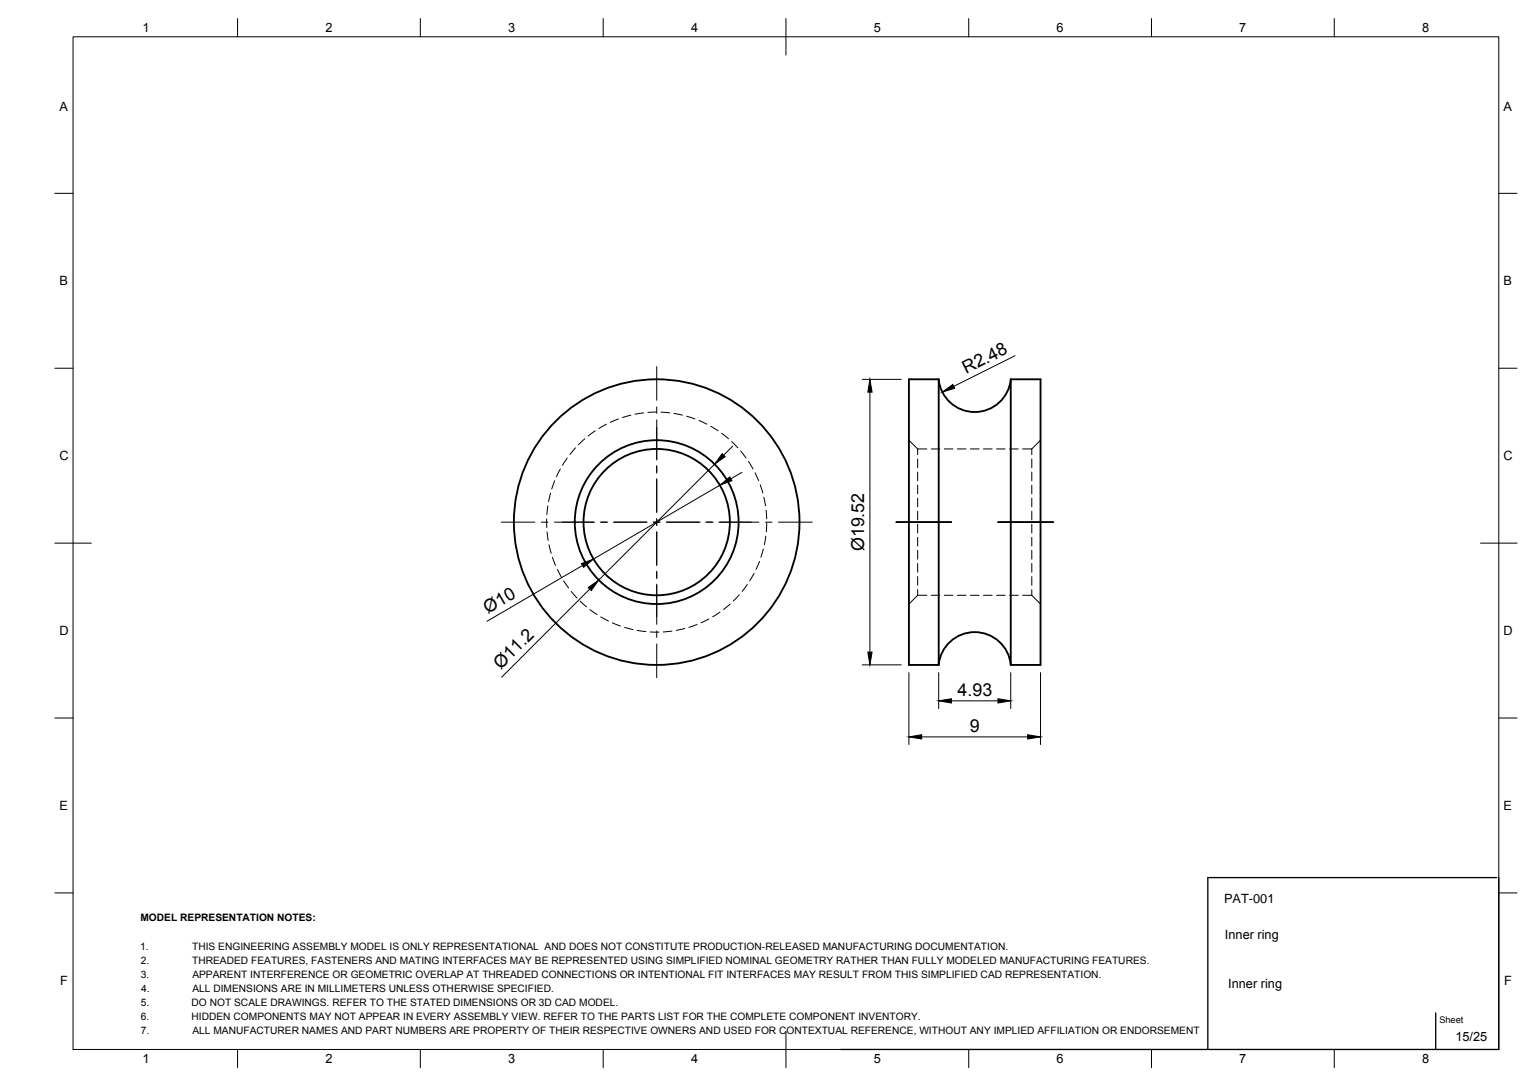
ISO-10303-21;
HEADER;
/* Generated by software containing ST-Developer
 * from STEP Tools, Inc. (www.steptools.com) 
 */

FILE_DESCRIPTION(
/* description */ ('PAT-001'),
/* implementation_level */ '2;1');

FILE_NAME(
/* name */ 'Inner ring.step',
/* time_stamp */ '2026-10-29T17:07:15-07:00',
/* author */ (''),
/* organization */ (''),
/* preprocessor_version */ 'ST-DEVELOPER v20.2',
/* originating_system */ 'Autodesk Translation Framework v15.17.0.0',
/* authorisation */ '');

FILE_SCHEMA (('AUTOMOTIVE_DESIGN { 1 0 10303 214 3 1 1 }'));
ENDSEC;

DATA;
#10=MECHANICAL_DESIGN_GEOMETRIC_PRESENTATION_REPRESENTATION('',(#378),#9622);
#305=CONICAL_SURFACE('',#5582,0.53,0.785398163397448);
#306=CONICAL_SURFACE('',#5589,0.53,0.785398163397448);
#321=TOROIDAL_SURFACE('',#5571,1.,0.247676);
#328=SHAPE_REPRESENTATION_RELATIONSHIP('SRR','None',#9752,#353);
#353=ADVANCED_BREP_SHAPE_REPRESENTATION('',(#411),#9601);
#378=STYLED_ITEM('',(#9962),#411);
#411=MANIFOLD_SOLID_BREP('Body1',#5203);
#449=FACE_BOUND('',#1055,.T.);
#450=FACE_BOUND('',#1058,.T.);
#542=PLANE('',#5584);
#543=PLANE('',#5587);
#742=FACE_OUTER_BOUND('',#1050,.T.);
#743=FACE_OUTER_BOUND('',#1051,.T.);
#744=FACE_OUTER_BOUND('',#1052,.T.);
#745=FACE_OUTER_BOUND('',#1053,.T.);
#746=FACE_OUTER_BOUND('',#1054,.T.);
#747=FACE_OUTER_BOUND('',#1056,.T.);
#748=FACE_OUTER_BOUND('',#1057,.T.);
#749=FACE_OUTER_BOUND('',#1059,.T.);
#1050=EDGE_LOOP('',(#3595,#3596,#3597,#3598,#3599,#3600));
#1051=EDGE_LOOP('',(#3601,#3602,#3603,#3604,#3605));
#1052=EDGE_LOOP('',(#3606,#3607,#3608,#3609));
#1053=EDGE_LOOP('',(#3610,#3611,#3612,#3613));
#1054=EDGE_LOOP('',(#3614));
#1055=EDGE_LOOP('',(#3615));
#1056=EDGE_LOOP('',(#3616,#3617,#3618,#3619,#3620));
#1057=EDGE_LOOP('',(#3621));
#1058=EDGE_LOOP('',(#3622));
#1059=EDGE_LOOP('',(#3623,#3624,#3625,#3626));
#1411=LINE('',#7821,#1816);
#1412=LINE('',#7827,#1817);
#1413=LINE('',#7831,#1818);
#1414=LINE('',#7837,#1819);
#1415=LINE('',#7842,#1820);
#1816=VECTOR('',#6258,0.976185);
#1817=VECTOR('',#6265,0.5);
#1818=VECTOR('',#6270,0.53);
#1819=VECTOR('',#6279,0.976185);
#1820=VECTOR('',#6286,0.53);
#2234=CIRCLE('',#5572,0.976185);
#2235=CIRCLE('',#5573,0.976185);
#2236=CIRCLE('',#5574,0.247676);
#2237=CIRCLE('',#5575,0.976185);
#2238=CIRCLE('',#5576,0.976185);
#2239=CIRCLE('',#5578,0.976185);
#2240=CIRCLE('',#5580,0.5);
#2241=CIRCLE('',#5581,0.5);
#2242=CIRCLE('',#5583,0.56);
#2243=CIRCLE('',#5586,0.976185);
#2244=CIRCLE('',#5588,0.56);
#2446=VERTEX_POINT('',#7810);
#2447=VERTEX_POINT('',#7811);
#2448=VERTEX_POINT('',#7814);
#2449=VERTEX_POINT('',#7816);
#2450=VERTEX_POINT('',#7820);
#2451=VERTEX_POINT('',#7824);
#2452=VERTEX_POINT('',#7826);
#2453=VERTEX_POINT('',#7830);
#2454=VERTEX_POINT('',#7835);
#2455=VERTEX_POINT('',#7839);
#2901=EDGE_CURVE('',#2446,#2447,#2234,.T.);
#2902=EDGE_CURVE('',#2447,#2446,#2235,.T.);
#2903=EDGE_CURVE('',#2447,#2448,#2236,.T.);
#2904=EDGE_CURVE('',#2449,#2448,#2237,.T.);
#2905=EDGE_CURVE('',#2448,#2449,#2238,.T.);
#2906=EDGE_CURVE('',#2449,#2450,#1411,.T.);
#2907=EDGE_CURVE('',#2450,#2450,#2239,.T.);
#2908=EDGE_CURVE('',#2451,#2451,#2240,.T.);
#2909=EDGE_CURVE('',#2451,#2452,#1412,.T.);
#2910=EDGE_CURVE('',#2452,#2452,#2241,.T.);
#2911=EDGE_CURVE('',#2452,#2453,#1413,.T.);
#2912=EDGE_CURVE('',#2453,#2453,#2242,.T.);
#2913=EDGE_CURVE('',#2454,#2454,#2243,.T.);
#2914=EDGE_CURVE('',#2454,#2446,#1414,.T.);
#2915=EDGE_CURVE('',#2455,#2455,#2244,.T.);
#2916=EDGE_CURVE('',#2455,#2451,#1415,.T.);
#3595=ORIENTED_EDGE('',*,*,#2901,.F.);
#3596=ORIENTED_EDGE('',*,*,#2902,.F.);
#3597=ORIENTED_EDGE('',*,*,#2903,.T.);
#3598=ORIENTED_EDGE('',*,*,#2904,.F.);
#3599=ORIENTED_EDGE('',*,*,#2905,.F.);
#3600=ORIENTED_EDGE('',*,*,#2903,.F.);
#3601=ORIENTED_EDGE('',*,*,#2904,.T.);
#3602=ORIENTED_EDGE('',*,*,#2905,.T.);
#3603=ORIENTED_EDGE('',*,*,#2906,.T.);
#3604=ORIENTED_EDGE('',*,*,#2907,.T.);
#3605=ORIENTED_EDGE('',*,*,#2906,.F.);
#3606=ORIENTED_EDGE('',*,*,#2908,.T.);
#3607=ORIENTED_EDGE('',*,*,#2909,.T.);
#3608=ORIENTED_EDGE('',*,*,#2910,.F.);
#3609=ORIENTED_EDGE('',*,*,#2909,.F.);
#3610=ORIENTED_EDGE('',*,*,#2910,.T.);
#3611=ORIENTED_EDGE('',*,*,#2911,.T.);
#3612=ORIENTED_EDGE('',*,*,#2912,.F.);
#3613=ORIENTED_EDGE('',*,*,#2911,.F.);
#3614=ORIENTED_EDGE('',*,*,#2907,.F.);
#3615=ORIENTED_EDGE('',*,*,#2912,.T.);
#3616=ORIENTED_EDGE('',*,*,#2913,.F.);
#3617=ORIENTED_EDGE('',*,*,#2914,.T.);
#3618=ORIENTED_EDGE('',*,*,#2901,.T.);
#3619=ORIENTED_EDGE('',*,*,#2902,.T.);
#3620=ORIENTED_EDGE('',*,*,#2914,.F.);
#3621=ORIENTED_EDGE('',*,*,#2913,.T.);
#3622=ORIENTED_EDGE('',*,*,#2915,.F.);
#3623=ORIENTED_EDGE('',*,*,#2915,.T.);
#3624=ORIENTED_EDGE('',*,*,#2916,.T.);
#3625=ORIENTED_EDGE('',*,*,#2908,.F.);
#3626=ORIENTED_EDGE('',*,*,#2916,.F.);
#4840=CYLINDRICAL_SURFACE('',#5577,0.976185);
#4841=CYLINDRICAL_SURFACE('',#5579,0.5);
#4842=CYLINDRICAL_SURFACE('',#5585,0.976185);
#4929=ADVANCED_FACE('',(#742),#321,.F.);
#4930=ADVANCED_FACE('',(#743),#4840,.T.);
#4931=ADVANCED_FACE('',(#744),#4841,.F.);
#4932=ADVANCED_FACE('',(#745),#305,.F.);
#4933=ADVANCED_FACE('',(#746,#449),#542,.T.);
#4934=ADVANCED_FACE('',(#747),#4842,.T.);
#4935=ADVANCED_FACE('',(#748,#450),#543,.T.);
#4936=ADVANCED_FACE('',(#749),#306,.F.);
#5203=CLOSED_SHELL('',(#4929,#4930,#4931,#4932,#4933,#4934,#4935,#4936));
#5570=AXIS2_PLACEMENT_3D('',#7808,#6242,#6243);
#5571=AXIS2_PLACEMENT_3D('',#7809,#6244,#6245);
#5572=AXIS2_PLACEMENT_3D('',#7812,#6246,#6247);
#5573=AXIS2_PLACEMENT_3D('',#7813,#6248,#6249);
#5574=AXIS2_PLACEMENT_3D('',#7815,#6250,#6251);
#5575=AXIS2_PLACEMENT_3D('',#7817,#6252,#6253);
#5576=AXIS2_PLACEMENT_3D('',#7818,#6254,#6255);
#5577=AXIS2_PLACEMENT_3D('',#7819,#6256,#6257);
#5578=AXIS2_PLACEMENT_3D('',#7822,#6259,#6260);
#5579=AXIS2_PLACEMENT_3D('',#7823,#6261,#6262);
#5580=AXIS2_PLACEMENT_3D('',#7825,#6263,#6264);
#5581=AXIS2_PLACEMENT_3D('',#7828,#6266,#6267);
#5582=AXIS2_PLACEMENT_3D('',#7829,#6268,#6269);
#5583=AXIS2_PLACEMENT_3D('',#7832,#6271,#6272);
#5584=AXIS2_PLACEMENT_3D('',#7833,#6273,#6274);
#5585=AXIS2_PLACEMENT_3D('',#7834,#6275,#6276);
#5586=AXIS2_PLACEMENT_3D('',#7836,#6277,#6278);
#5587=AXIS2_PLACEMENT_3D('',#7838,#6280,#6281);
#5588=AXIS2_PLACEMENT_3D('',#7840,#6282,#6283);
#5589=AXIS2_PLACEMENT_3D('',#7841,#6284,#6285);
#6242=DIRECTION('axis',(0.,0.,1.));
#6243=DIRECTION('refdir',(1.,0.,0.));
#6244=DIRECTION('center_axis',(0.,-1.,0.));
#6245=DIRECTION('ref_axis',(0.,0.,-1.));
#6246=DIRECTION('center_axis',(0.,-1.,0.));
#6247=DIRECTION('ref_axis',(1.,0.,0.));
#6248=DIRECTION('center_axis',(0.,-1.,0.));
#6249=DIRECTION('ref_axis',(1.,0.,0.));
#6250=DIRECTION('center_axis',(1.,0.,1.22464679914735E-16));
#6251=DIRECTION('ref_axis',(-1.22464679914735E-16,0.,1.));
#6252=DIRECTION('center_axis',(0.,1.,0.));
#6253=DIRECTION('ref_axis',(1.,0.,0.));
#6254=DIRECTION('center_axis',(0.,1.,0.));
#6255=DIRECTION('ref_axis',(1.,0.,0.));
#6256=DIRECTION('center_axis',(0.,-1.,0.));
#6257=DIRECTION('ref_axis',(1.,0.,0.));
#6258=DIRECTION('',(0.,1.,0.));
#6259=DIRECTION('center_axis',(0.,-1.,0.));
#6260=DIRECTION('ref_axis',(1.,0.,0.));
#6261=DIRECTION('center_axis',(0.,-1.,0.));
#6262=DIRECTION('ref_axis',(1.,0.,0.));
#6263=DIRECTION('center_axis',(0.,-1.,0.));
#6264=DIRECTION('ref_axis',(1.,0.,0.));
#6265=DIRECTION('',(0.,1.,0.));
#6266=DIRECTION('center_axis',(0.,-1.,0.));
#6267=DIRECTION('ref_axis',(1.,0.,0.));
#6268=DIRECTION('center_axis',(0.,1.,0.));
#6269=DIRECTION('ref_axis',(1.,0.,0.));
#6270=DIRECTION('',(-0.707106781186547,0.707106781186548,-8.65956056235493E-17));
#6271=DIRECTION('center_axis',(0.,-1.,0.));
#6272=DIRECTION('ref_axis',(1.,0.,0.));
#6273=DIRECTION('center_axis',(0.,1.,0.));
#6274=DIRECTION('ref_axis',(0.,0.,1.));
#6275=DIRECTION('center_axis',(0.,-1.,0.));
#6276=DIRECTION('ref_axis',(1.,0.,0.));
#6277=DIRECTION('center_axis',(0.,-1.,0.));
#6278=DIRECTION('ref_axis',(1.,0.,0.));
#6279=DIRECTION('',(0.,1.,0.));
#6280=DIRECTION('center_axis',(0.,-1.,0.));
#6281=DIRECTION('ref_axis',(0.,0.,-1.));
#6282=DIRECTION('center_axis',(0.,-1.,0.));
#6283=DIRECTION('ref_axis',(1.,0.,0.));
#6284=DIRECTION('center_axis',(0.,-1.,0.));
#6285=DIRECTION('ref_axis',(1.,0.,0.));
#6286=DIRECTION('',(0.707106781186547,0.707106781186548,8.65956056235493E-17));
#7808=CARTESIAN_POINT('',(0.,0.,0.));
#7809=CARTESIAN_POINT('Origin',(0.,0.,0.));
#7810=CARTESIAN_POINT('',(-0.976185,-0.246528389340863,-1.19548183562566E-16));
#7811=CARTESIAN_POINT('',(-1.19548183562566E-16,-0.246528389340863,0.976185));
#7812=CARTESIAN_POINT('Origin',(0.,-0.246528389340863,0.));
#7813=CARTESIAN_POINT('Origin',(0.,-0.246528389340863,0.));
#7814=CARTESIAN_POINT('',(-1.19548183562566E-16,0.246528389340863,0.976185));
#7815=CARTESIAN_POINT('Origin',(-1.22464679914735E-16,0.,1.));
#7816=CARTESIAN_POINT('',(-0.976185,0.246528389340863,1.19548183562566E-16));
#7817=CARTESIAN_POINT('Origin',(0.,0.246528389340863,0.));
#7818=CARTESIAN_POINT('Origin',(0.,0.246528389340863,0.));
#7819=CARTESIAN_POINT('Origin',(0.,0.,0.));
#7820=CARTESIAN_POINT('',(-0.976185,0.45,-1.19548183562566E-16));
#7821=CARTESIAN_POINT('',(-0.976185,0.,-1.19548183562566E-16));
#7822=CARTESIAN_POINT('Origin',(0.,0.45,0.));
#7823=CARTESIAN_POINT('Origin',(0.,0.,0.));
#7824=CARTESIAN_POINT('',(-0.5,-0.39,-6.12323399573677E-17));
#7825=CARTESIAN_POINT('Origin',(0.,-0.39,0.));
#7826=CARTESIAN_POINT('',(-0.5,0.39,-6.12323399573677E-17));
#7827=CARTESIAN_POINT('',(-0.5,0.,-6.12323399573677E-17));
#7828=CARTESIAN_POINT('Origin',(0.,0.39,0.));
#7829=CARTESIAN_POINT('Origin',(0.,0.42,0.));
#7830=CARTESIAN_POINT('',(-0.56,0.45,-6.85802207522518E-17));
#7831=CARTESIAN_POINT('',(-0.53,0.42,-6.49062803548097E-17));
#7832=CARTESIAN_POINT('Origin',(0.,0.45,0.));
#7833=CARTESIAN_POINT('Origin',(0.976185,0.45,0.));
#7834=CARTESIAN_POINT('Origin',(0.,0.,0.));
#7835=CARTESIAN_POINT('',(-0.976185,-0.45,-1.19548183562566E-16));
#7836=CARTESIAN_POINT('Origin',(0.,-0.45,0.));
#7837=CARTESIAN_POINT('',(-0.976185,0.,-1.19548183562566E-16));
#7838=CARTESIAN_POINT('Origin',(0.56,-0.45,0.));
#7839=CARTESIAN_POINT('',(-0.56,-0.45,-6.85802207522518E-17));
#7840=CARTESIAN_POINT('Origin',(0.,-0.45,0.));
#7841=CARTESIAN_POINT('Origin',(0.,-0.42,0.));
#7842=CARTESIAN_POINT('',(-0.53,-0.42,-6.49062803548097E-17));
#9571=UNCERTAINTY_MEASURE_WITH_UNIT(LENGTH_MEASURE(0.001),#9623,
'DISTANCE_ACCURACY_VALUE',
'Maximum model space distance between geometric entities at asserted c
onnectivities');
#9592=UNCERTAINTY_MEASURE_WITH_UNIT(LENGTH_MEASURE(0.001),#9623,
'DISTANCE_ACCURACY_VALUE',
'Maximum model space distance between geometric entities at asserted c
onnectivities');
#9601=(
GEOMETRIC_REPRESENTATION_CONTEXT(3)
GLOBAL_UNCERTAINTY_ASSIGNED_CONTEXT((#9571))
GLOBAL_UNIT_ASSIGNED_CONTEXT((#9623,#9625,#9626))
REPRESENTATION_CONTEXT('','3D')
);
#9622=(
GEOMETRIC_REPRESENTATION_CONTEXT(3)
GLOBAL_UNCERTAINTY_ASSIGNED_CONTEXT((#9592))
GLOBAL_UNIT_ASSIGNED_CONTEXT((#9623,#9625,#9626))
REPRESENTATION_CONTEXT('','3D')
);
#9623=(
LENGTH_UNIT()
NAMED_UNIT(*)
SI_UNIT(.CENTI.,.METRE.)
);
#9625=(
NAMED_UNIT(*)
PLANE_ANGLE_UNIT()
SI_UNIT($,.RADIAN.)
);
#9626=(
NAMED_UNIT(*)
SI_UNIT($,.STERADIAN.)
SOLID_ANGLE_UNIT()
);
#9635=SHAPE_DEFINITION_REPRESENTATION(#9664,#9752);
#9664=PRODUCT_DEFINITION_SHAPE('',$,#9782);
#9752=SHAPE_REPRESENTATION('',(#5570),#9601);
#9773=PRODUCT_DEFINITION_CONTEXT('part definition',#9862,'design');
#9782=PRODUCT_DEFINITION('Inner ring','Inner ring',#9811,#9773);
#9811=PRODUCT_DEFINITION_FORMATION('',$,#9872);
#9862=APPLICATION_CONTEXT(
'Core Data for Automotive Mechanical Design Process');
#9863=PRODUCT_CONTEXT('part definition',#9862,'mechanical');
#9872=PRODUCT('Inner ring','Inner ring','Inner ring',(#9863));
#9956=COLOUR_RGB('Grey',0.48,0.52,0.57);
#9957=FILL_AREA_STYLE_COLOUR('',#9956);
#9958=FILL_AREA_STYLE('',(#9957));
#9959=SURFACE_STYLE_FILL_AREA(#9958);
#9960=SURFACE_SIDE_STYLE('',(#9959));
#9961=SURFACE_STYLE_USAGE(.BOTH.,#9960);
#9962=PRESENTATION_STYLE_ASSIGNMENT((#9961));
ENDSEC;
END-ISO-10303-21;
